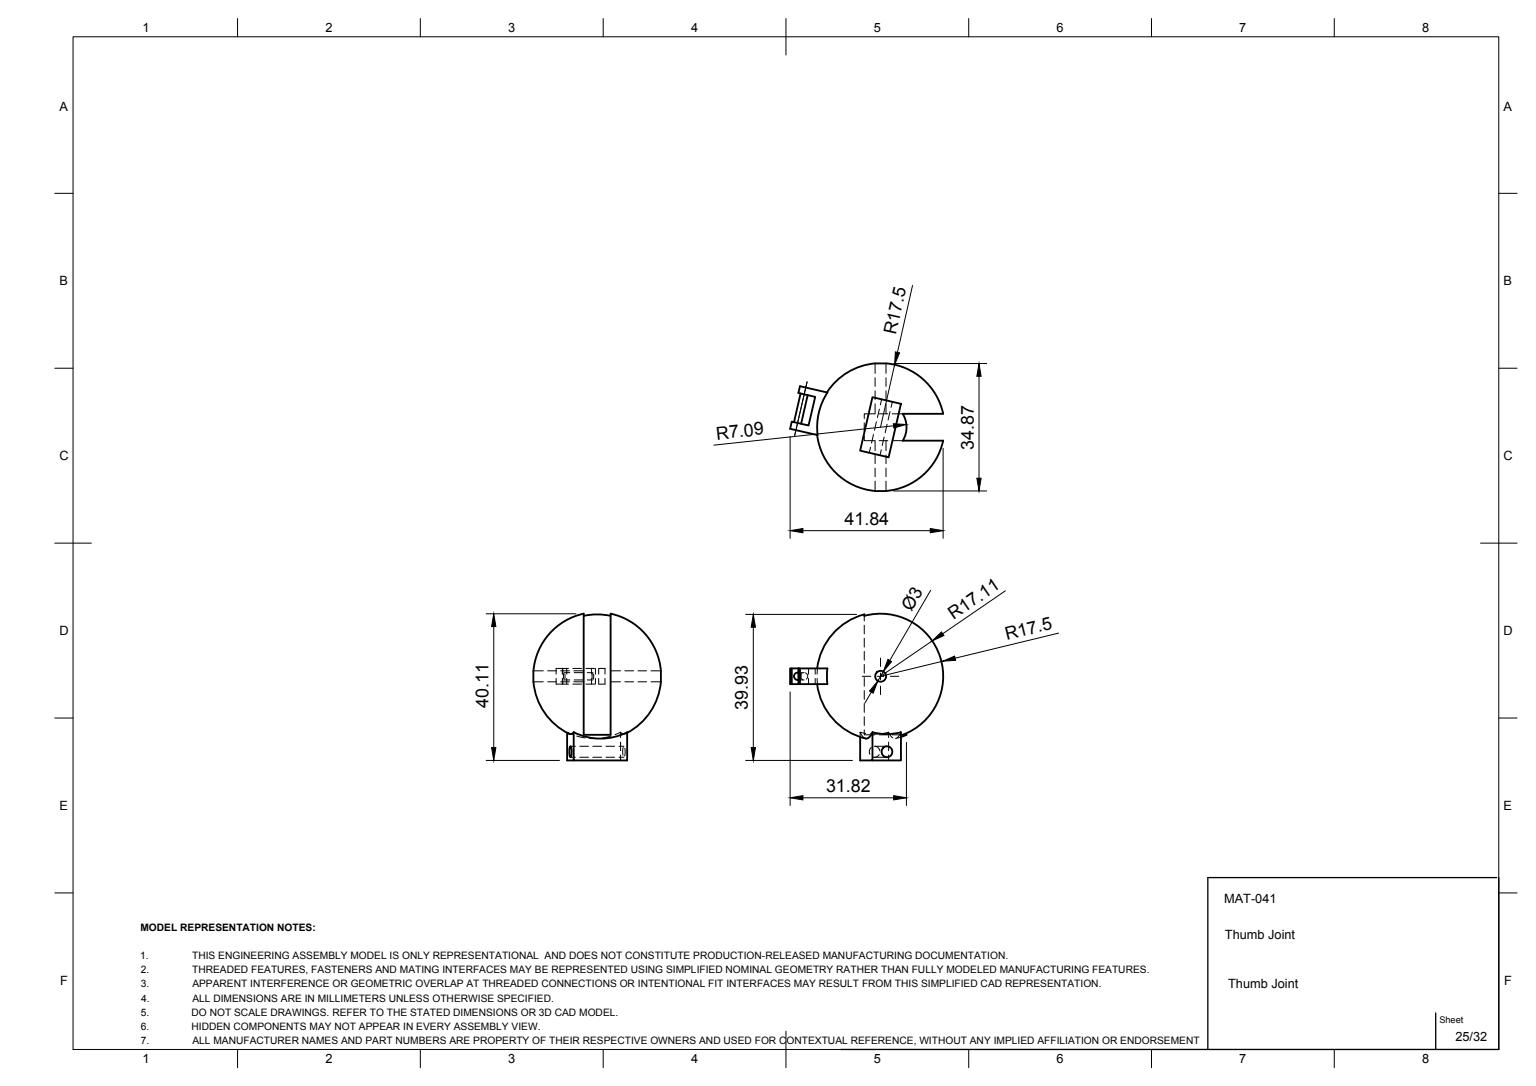
ISO-10303-21;
HEADER;
/* Generated by software containing ST-Developer
 * from STEP Tools, Inc. (www.steptools.com) 
 */

FILE_DESCRIPTION(
/* description */ ('STEP AP214'),
/* implementation_level */ '2;1');

FILE_NAME(
/* name */ 'Thumb Joint.step',
/* time_stamp */ '2026-11-14T21:57:47-08:00',
/* author */ (''),
/* organization */ (''),
/* preprocessor_version */ 'ST-DEVELOPER v20.2',
/* originating_system */ 'Autodesk Translation Framework v15.17.0.0',
/* authorisation */ '');

FILE_SCHEMA (('AUTOMOTIVE_DESIGN { 1 0 10303 214 3 1 1 }'));
ENDSEC;

DATA;
#10=MECHANICAL_DESIGN_GEOMETRIC_PRESENTATION_REPRESENTATION('',(#260),#13199);
#224=SHAPE_REPRESENTATION_RELATIONSHIP('SRR','None',#13296,#242);
#242=ADVANCED_BREP_SHAPE_REPRESENTATION('',(#278),#13192);
#260=STYLED_ITEM('',(#13410),#278);
#278=MANIFOLD_SOLID_BREP('Body1',#6855);
#354=FACE_BOUND('',#2551,.T.);
#355=FACE_BOUND('',#2552,.T.);
#356=FACE_BOUND('',#2556,.T.);
#357=FACE_BOUND('',#2559,.T.);
#358=FACE_BOUND('',#2562,.T.);
#359=FACE_BOUND('',#2565,.T.);
#360=FACE_BOUND('',#2574,.T.);
#361=FACE_BOUND('',#2576,.T.);
#543=PLANE('',#7648);
#544=PLANE('',#7649);
#545=PLANE('',#7650);
#546=PLANE('',#7651);
#547=PLANE('',#7652);
#548=PLANE('',#7653);
#549=PLANE('',#7654);
#550=PLANE('',#7655);
#551=PLANE('',#7656);
#552=PLANE('',#7657);
#553=PLANE('',#7658);
#554=PLANE('',#7659);
#555=PLANE('',#7660);
#556=PLANE('',#7661);
#557=PLANE('',#7662);
#558=PLANE('',#7663);
#559=PLANE('',#7664);
#560=PLANE('',#7665);
#980=LINE('',#12181,#1498);
#981=LINE('',#12187,#1499);
#982=LINE('',#12193,#1500);
#983=LINE('',#12199,#1501);
#984=LINE('',#12235,#1502);
#985=LINE('',#12237,#1503);
#986=LINE('',#12239,#1504);
#987=LINE('',#12240,#1505);
#988=LINE('',#12243,#1506);
#989=LINE('',#12245,#1507);
#990=LINE('',#12246,#1508);
#991=LINE('',#12249,#1509);
#992=LINE('',#12250,#1510);
#993=LINE('',#12253,#1511);
#994=LINE('',#12254,#1512);
#995=LINE('',#12256,#1513);
#996=LINE('',#12260,#1514);
#997=LINE('',#12261,#1515);
#998=LINE('',#12264,#1516);
#999=LINE('',#12265,#1517);
#1000=LINE('',#12267,#1518);
#1001=LINE('',#12272,#1519);
#1002=LINE('',#12273,#1520);
#1003=LINE('',#12274,#1521);
#1004=LINE('',#12276,#1522);
#1005=LINE('',#12278,#1523);
#1006=LINE('',#12279,#1524);
#1007=LINE('',#12282,#1525);
#1008=LINE('',#12283,#1526);
#1009=LINE('',#12286,#1527);
#1010=LINE('',#12288,#1528);
#1011=LINE('',#12290,#1529);
#1012=LINE('',#12291,#1530);
#1013=LINE('',#12292,#1531);
#1014=LINE('',#12295,#1532);
#1015=LINE('',#12297,#1533);
#1016=LINE('',#12298,#1534);
#1498=VECTOR('',#9321,1.);
#1499=VECTOR('',#9328,1.5);
#1500=VECTOR('',#9335,1.5);
#1501=VECTOR('',#9342,1.5);
#1502=VECTOR('',#9381,1000.);
#1503=VECTOR('',#9382,1000.);
#1504=VECTOR('',#9383,1000.);
#1505=VECTOR('',#9384,1000.);
#1506=VECTOR('',#9387,1000.);
#1507=VECTOR('',#9388,1000.);
#1508=VECTOR('',#9389,1000.);
#1509=VECTOR('',#9392,1000.);
#1510=VECTOR('',#9393,1000.);
#1511=VECTOR('',#9396,1000.);
#1512=VECTOR('',#9397,1000.);
#1513=VECTOR('',#9400,1000.);
#1514=VECTOR('',#9405,1000.);
#1515=VECTOR('',#9406,1000.);
#1516=VECTOR('',#9409,1000.);
#1517=VECTOR('',#9410,1000.);
#1518=VECTOR('',#9413,1000.);
#1519=VECTOR('',#9418,1000.);
#1520=VECTOR('',#9419,1000.);
#1521=VECTOR('',#9420,1000.);
#1522=VECTOR('',#9421,1000.);
#1523=VECTOR('',#9422,1000.);
#1524=VECTOR('',#9423,1000.);
#1525=VECTOR('',#9426,1000.);
#1526=VECTOR('',#9427,1000.);
#1527=VECTOR('',#9430,1000.);
#1528=VECTOR('',#9431,1000.);
#1529=VECTOR('',#9432,1000.);
#1530=VECTOR('',#9433,1000.);
#1531=VECTOR('',#9434,1000.);
#1532=VECTOR('',#9439,1000.);
#1533=VECTOR('',#9442,1000.);
#1534=VECTOR('',#9443,1000.);
#1757=CYLINDRICAL_SURFACE('',#7619,1.);
#1758=CYLINDRICAL_SURFACE('',#7622,1.5);
#1759=CYLINDRICAL_SURFACE('',#7625,1.5);
#1760=CYLINDRICAL_SURFACE('',#7628,1.5);
#1799=SPHERICAL_SURFACE('',#7631,17.5);
#2085=FACE_OUTER_BOUND('',#2546,.T.);
#2086=FACE_OUTER_BOUND('',#2547,.T.);
#2087=FACE_OUTER_BOUND('',#2548,.T.);
#2088=FACE_OUTER_BOUND('',#2549,.T.);
#2089=FACE_OUTER_BOUND('',#2550,.T.);
#2090=FACE_OUTER_BOUND('',#2553,.T.);
#2091=FACE_OUTER_BOUND('',#2554,.T.);
#2092=FACE_OUTER_BOUND('',#2555,.T.);
#2093=FACE_OUTER_BOUND('',#2557,.T.);
#2094=FACE_OUTER_BOUND('',#2558,.T.);
#2095=FACE_OUTER_BOUND('',#2560,.T.);
#2096=FACE_OUTER_BOUND('',#2561,.T.);
#2097=FACE_OUTER_BOUND('',#2563,.T.);
#2098=FACE_OUTER_BOUND('',#2564,.T.);
#2099=FACE_OUTER_BOUND('',#2566,.T.);
#2100=FACE_OUTER_BOUND('',#2567,.T.);
#2101=FACE_OUTER_BOUND('',#2568,.T.);
#2102=FACE_OUTER_BOUND('',#2569,.T.);
#2103=FACE_OUTER_BOUND('',#2570,.T.);
#2104=FACE_OUTER_BOUND('',#2571,.T.);
#2105=FACE_OUTER_BOUND('',#2572,.T.);
#2106=FACE_OUTER_BOUND('',#2573,.T.);
#2107=FACE_OUTER_BOUND('',#2575,.T.);
#2546=EDGE_LOOP('',(#5910,#5911,#5912,#5913));
#2547=EDGE_LOOP('',(#5914,#5915,#5916,#5917));
#2548=EDGE_LOOP('',(#5918,#5919,#5920,#5921));
#2549=EDGE_LOOP('',(#5922,#5923,#5924,#5925));
#2550=EDGE_LOOP('',(#5926,#5927,#5928,#5929,#5930,#5931,#5932,#5933,#5934,
#5935,#5936,#5937));
#2551=EDGE_LOOP('',(#5938,#5939,#5940,#5941));
#2552=EDGE_LOOP('',(#5942,#5943,#5944,#5945));
#2553=EDGE_LOOP('',(#5946,#5947,#5948,#5949));
#2554=EDGE_LOOP('',(#5950,#5951,#5952,#5953));
#2555=EDGE_LOOP('',(#5954,#5955,#5956,#5957));
#2556=EDGE_LOOP('',(#5958));
#2557=EDGE_LOOP('',(#5959,#5960,#5961,#5962));
#2558=EDGE_LOOP('',(#5963,#5964,#5965,#5966));
#2559=EDGE_LOOP('',(#5967));
#2560=EDGE_LOOP('',(#5968,#5969,#5970,#5971));
#2561=EDGE_LOOP('',(#5972,#5973,#5974,#5975));
#2562=EDGE_LOOP('',(#5976));
#2563=EDGE_LOOP('',(#5977,#5978,#5979,#5980));
#2564=EDGE_LOOP('',(#5981,#5982,#5983,#5984));
#2565=EDGE_LOOP('',(#5985));
#2566=EDGE_LOOP('',(#5986,#5987,#5988,#5989));
#2567=EDGE_LOOP('',(#5990,#5991,#5992,#5993,#5994,#5995,#5996,#5997));
#2568=EDGE_LOOP('',(#5998,#5999,#6000,#6001));
#2569=EDGE_LOOP('',(#6002,#6003,#6004,#6005,#6006,#6007,#6008,#6009));
#2570=EDGE_LOOP('',(#6010,#6011,#6012,#6013));
#2571=EDGE_LOOP('',(#6014,#6015,#6016,#6017));
#2572=EDGE_LOOP('',(#6018,#6019,#6020,#6021));
#2573=EDGE_LOOP('',(#6022,#6023,#6024,#6025));
#2574=EDGE_LOOP('',(#6026));
#2575=EDGE_LOOP('',(#6027,#6028,#6029,#6030));
#2576=EDGE_LOOP('',(#6031));
#2915=CIRCLE('',#7620,1.);
#2916=CIRCLE('',#7621,1.);
#2917=CIRCLE('',#7623,1.5);
#2918=CIRCLE('',#7624,1.5);
#2919=CIRCLE('',#7626,1.5);
#2920=CIRCLE('',#7627,1.5);
#2921=CIRCLE('',#7629,1.5);
#2922=CIRCLE('',#7630,1.5);
#2923=CIRCLE('',#7632,17.5);
#2924=CIRCLE('',#7633,17.1097742533325);
#2925=CIRCLE('',#7634,7.08872343937892);
#2926=CIRCLE('',#7635,17.1097742533325);
#2927=CIRCLE('',#7636,17.5);
#2928=CIRCLE('',#7637,17.1097742533325);
#2929=CIRCLE('',#7638,16.9253361239603);
#2930=CIRCLE('',#7639,17.1097742533325);
#2931=CIRCLE('',#7640,17.3675981074726);
#2932=CIRCLE('',#7641,16.4471056942753);
#2933=CIRCLE('',#7642,17.3675981074726);
#2934=CIRCLE('',#7643,16.4471056942753);
#2935=CIRCLE('',#7644,17.0367250374008);
#2936=CIRCLE('',#7645,15.8113883008419);
#2937=CIRCLE('',#7646,17.0367250374008);
#2938=CIRCLE('',#7647,15.8113883008419);
#3439=VERTEX_POINT('',#12178);
#3440=VERTEX_POINT('',#12180);
#3441=VERTEX_POINT('',#12184);
#3442=VERTEX_POINT('',#12186);
#3443=VERTEX_POINT('',#12190);
#3444=VERTEX_POINT('',#12192);
#3445=VERTEX_POINT('',#12196);
#3446=VERTEX_POINT('',#12198);
#3447=VERTEX_POINT('',#12202);
#3448=VERTEX_POINT('',#12204);
#3449=VERTEX_POINT('',#12206);
#3450=VERTEX_POINT('',#12208);
#3451=VERTEX_POINT('',#12211);
#3452=VERTEX_POINT('',#12213);
#3453=VERTEX_POINT('',#12216);
#3454=VERTEX_POINT('',#12217);
#3455=VERTEX_POINT('',#12219);
#3456=VERTEX_POINT('',#12221);
#3457=VERTEX_POINT('',#12224);
#3458=VERTEX_POINT('',#12225);
#3459=VERTEX_POINT('',#12227);
#3460=VERTEX_POINT('',#12229);
#3461=VERTEX_POINT('',#12233);
#3462=VERTEX_POINT('',#12234);
#3463=VERTEX_POINT('',#12236);
#3464=VERTEX_POINT('',#12238);
#3465=VERTEX_POINT('',#12242);
#3466=VERTEX_POINT('',#12244);
#3467=VERTEX_POINT('',#12248);
#3468=VERTEX_POINT('',#12252);
#3469=VERTEX_POINT('',#12259);
#3470=VERTEX_POINT('',#12263);
#3471=VERTEX_POINT('',#12270);
#3472=VERTEX_POINT('',#12271);
#3473=VERTEX_POINT('',#12275);
#3474=VERTEX_POINT('',#12277);
#3475=VERTEX_POINT('',#12281);
#3476=VERTEX_POINT('',#12285);
#3477=VERTEX_POINT('',#12287);
#3478=VERTEX_POINT('',#12289);
#4292=EDGE_CURVE('',#3439,#3439,#2915,.T.);
#4293=EDGE_CURVE('',#3439,#3440,#980,.T.);
#4294=EDGE_CURVE('',#3440,#3440,#2916,.T.);
#4295=EDGE_CURVE('',#3441,#3441,#2917,.T.);
#4296=EDGE_CURVE('',#3441,#3442,#981,.T.);
#4297=EDGE_CURVE('',#3442,#3442,#2918,.T.);
#4298=EDGE_CURVE('',#3443,#3443,#2919,.T.);
#4299=EDGE_CURVE('',#3443,#3444,#982,.T.);
#4300=EDGE_CURVE('',#3444,#3444,#2920,.T.);
#4301=EDGE_CURVE('',#3445,#3445,#2921,.T.);
#4302=EDGE_CURVE('',#3445,#3446,#983,.T.);
#4303=EDGE_CURVE('',#3446,#3446,#2922,.T.);
#4304=EDGE_CURVE('',#3444,#3447,#2923,.T.);
#4305=EDGE_CURVE('',#3448,#3447,#2924,.T.);
#4306=EDGE_CURVE('',#3449,#3448,#2925,.T.);
#4307=EDGE_CURVE('',#3450,#3449,#2926,.T.);
#4308=EDGE_CURVE('',#3450,#3445,#2927,.T.);
#4309=EDGE_CURVE('',#3451,#3450,#2928,.T.);
#4310=EDGE_CURVE('',#3452,#3451,#2929,.T.);
#4311=EDGE_CURVE('',#3447,#3452,#2930,.T.);
#4312=EDGE_CURVE('',#3453,#3454,#2931,.T.);
#4313=EDGE_CURVE('',#3455,#3453,#2932,.T.);
#4314=EDGE_CURVE('',#3456,#3455,#2933,.T.);
#4315=EDGE_CURVE('',#3454,#3456,#2934,.T.);
#4316=EDGE_CURVE('',#3457,#3458,#2935,.T.);
#4317=EDGE_CURVE('',#3458,#3459,#2936,.T.);
#4318=EDGE_CURVE('',#3460,#3459,#2937,.T.);
#4319=EDGE_CURVE('',#3457,#3460,#2938,.T.);
#4320=EDGE_CURVE('',#3461,#3462,#984,.T.);
#4321=EDGE_CURVE('',#3461,#3463,#985,.T.);
#4322=EDGE_CURVE('',#3463,#3464,#986,.T.);
#4323=EDGE_CURVE('',#3464,#3462,#987,.T.);
#4324=EDGE_CURVE('',#3465,#3457,#988,.T.);
#4325=EDGE_CURVE('',#3465,#3466,#989,.T.);
#4326=EDGE_CURVE('',#3466,#3458,#990,.T.);
#4327=EDGE_CURVE('',#3467,#3460,#991,.T.);
#4328=EDGE_CURVE('',#3465,#3467,#992,.T.);
#4329=EDGE_CURVE('',#3468,#3459,#993,.T.);
#4330=EDGE_CURVE('',#3467,#3468,#994,.T.);
#4331=EDGE_CURVE('',#3466,#3468,#995,.T.);
#4332=EDGE_CURVE('',#3452,#3469,#996,.T.);
#4333=EDGE_CURVE('',#3448,#3469,#997,.T.);
#4334=EDGE_CURVE('',#3451,#3470,#998,.T.);
#4335=EDGE_CURVE('',#3469,#3470,#999,.T.);
#4336=EDGE_CURVE('',#3470,#3449,#1000,.T.);
#4337=EDGE_CURVE('',#3471,#3472,#1001,.T.);
#4338=EDGE_CURVE('',#3472,#3462,#1002,.T.);
#4339=EDGE_CURVE('',#3464,#3456,#1003,.T.);
#4340=EDGE_CURVE('',#3473,#3455,#1004,.T.);
#4341=EDGE_CURVE('',#3474,#3473,#1005,.T.);
#4342=EDGE_CURVE('',#3474,#3471,#1006,.T.);
#4343=EDGE_CURVE('',#3475,#3453,#1007,.T.);
#4344=EDGE_CURVE('',#3473,#3475,#1008,.T.);
#4345=EDGE_CURVE('',#3476,#3461,#1009,.T.);
#4346=EDGE_CURVE('',#3477,#3476,#1010,.T.);
#4347=EDGE_CURVE('',#3478,#3477,#1011,.T.);
#4348=EDGE_CURVE('',#3475,#3478,#1012,.T.);
#4349=EDGE_CURVE('',#3463,#3454,#1013,.T.);
#4350=EDGE_CURVE('',#3474,#3478,#1014,.T.);
#4351=EDGE_CURVE('',#3471,#3477,#1015,.T.);
#4352=EDGE_CURVE('',#3472,#3476,#1016,.T.);
#5910=ORIENTED_EDGE('',*,*,#4292,.F.);
#5911=ORIENTED_EDGE('',*,*,#4293,.T.);
#5912=ORIENTED_EDGE('',*,*,#4294,.T.);
#5913=ORIENTED_EDGE('',*,*,#4293,.F.);
#5914=ORIENTED_EDGE('',*,*,#4295,.F.);
#5915=ORIENTED_EDGE('',*,*,#4296,.T.);
#5916=ORIENTED_EDGE('',*,*,#4297,.T.);
#5917=ORIENTED_EDGE('',*,*,#4296,.F.);
#5918=ORIENTED_EDGE('',*,*,#4298,.F.);
#5919=ORIENTED_EDGE('',*,*,#4299,.T.);
#5920=ORIENTED_EDGE('',*,*,#4300,.T.);
#5921=ORIENTED_EDGE('',*,*,#4299,.F.);
#5922=ORIENTED_EDGE('',*,*,#4301,.T.);
#5923=ORIENTED_EDGE('',*,*,#4302,.T.);
#5924=ORIENTED_EDGE('',*,*,#4303,.F.);
#5925=ORIENTED_EDGE('',*,*,#4302,.F.);
#5926=ORIENTED_EDGE('',*,*,#4300,.F.);
#5927=ORIENTED_EDGE('',*,*,#4304,.T.);
#5928=ORIENTED_EDGE('',*,*,#4305,.F.);
#5929=ORIENTED_EDGE('',*,*,#4306,.F.);
#5930=ORIENTED_EDGE('',*,*,#4307,.F.);
#5931=ORIENTED_EDGE('',*,*,#4308,.T.);
#5932=ORIENTED_EDGE('',*,*,#4301,.F.);
#5933=ORIENTED_EDGE('',*,*,#4308,.F.);
#5934=ORIENTED_EDGE('',*,*,#4309,.F.);
#5935=ORIENTED_EDGE('',*,*,#4310,.F.);
#5936=ORIENTED_EDGE('',*,*,#4311,.F.);
#5937=ORIENTED_EDGE('',*,*,#4304,.F.);
#5938=ORIENTED_EDGE('',*,*,#4312,.F.);
#5939=ORIENTED_EDGE('',*,*,#4313,.F.);
#5940=ORIENTED_EDGE('',*,*,#4314,.F.);
#5941=ORIENTED_EDGE('',*,*,#4315,.F.);
#5942=ORIENTED_EDGE('',*,*,#4316,.T.);
#5943=ORIENTED_EDGE('',*,*,#4317,.T.);
#5944=ORIENTED_EDGE('',*,*,#4318,.F.);
#5945=ORIENTED_EDGE('',*,*,#4319,.F.);
#5946=ORIENTED_EDGE('',*,*,#4320,.F.);
#5947=ORIENTED_EDGE('',*,*,#4321,.T.);
#5948=ORIENTED_EDGE('',*,*,#4322,.T.);
#5949=ORIENTED_EDGE('',*,*,#4323,.T.);
#5950=ORIENTED_EDGE('',*,*,#4316,.F.);
#5951=ORIENTED_EDGE('',*,*,#4324,.F.);
#5952=ORIENTED_EDGE('',*,*,#4325,.T.);
#5953=ORIENTED_EDGE('',*,*,#4326,.T.);
#5954=ORIENTED_EDGE('',*,*,#4324,.T.);
#5955=ORIENTED_EDGE('',*,*,#4319,.T.);
#5956=ORIENTED_EDGE('',*,*,#4327,.F.);
#5957=ORIENTED_EDGE('',*,*,#4328,.F.);
#5958=ORIENTED_EDGE('',*,*,#4295,.T.);
#5959=ORIENTED_EDGE('',*,*,#4327,.T.);
#5960=ORIENTED_EDGE('',*,*,#4318,.T.);
#5961=ORIENTED_EDGE('',*,*,#4329,.F.);
#5962=ORIENTED_EDGE('',*,*,#4330,.F.);
#5963=ORIENTED_EDGE('',*,*,#4317,.F.);
#5964=ORIENTED_EDGE('',*,*,#4326,.F.);
#5965=ORIENTED_EDGE('',*,*,#4331,.T.);
#5966=ORIENTED_EDGE('',*,*,#4329,.T.);
#5967=ORIENTED_EDGE('',*,*,#4297,.F.);
#5968=ORIENTED_EDGE('',*,*,#4325,.F.);
#5969=ORIENTED_EDGE('',*,*,#4328,.T.);
#5970=ORIENTED_EDGE('',*,*,#4330,.T.);
#5971=ORIENTED_EDGE('',*,*,#4331,.F.);
#5972=ORIENTED_EDGE('',*,*,#4305,.T.);
#5973=ORIENTED_EDGE('',*,*,#4311,.T.);
#5974=ORIENTED_EDGE('',*,*,#4332,.T.);
#5975=ORIENTED_EDGE('',*,*,#4333,.F.);
#5976=ORIENTED_EDGE('',*,*,#4298,.T.);
#5977=ORIENTED_EDGE('',*,*,#4310,.T.);
#5978=ORIENTED_EDGE('',*,*,#4334,.T.);
#5979=ORIENTED_EDGE('',*,*,#4335,.F.);
#5980=ORIENTED_EDGE('',*,*,#4332,.F.);
#5981=ORIENTED_EDGE('',*,*,#4309,.T.);
#5982=ORIENTED_EDGE('',*,*,#4307,.T.);
#5983=ORIENTED_EDGE('',*,*,#4336,.F.);
#5984=ORIENTED_EDGE('',*,*,#4334,.F.);
#5985=ORIENTED_EDGE('',*,*,#4303,.T.);
#5986=ORIENTED_EDGE('',*,*,#4306,.T.);
#5987=ORIENTED_EDGE('',*,*,#4333,.T.);
#5988=ORIENTED_EDGE('',*,*,#4335,.T.);
#5989=ORIENTED_EDGE('',*,*,#4336,.T.);
#5990=ORIENTED_EDGE('',*,*,#4337,.T.);
#5991=ORIENTED_EDGE('',*,*,#4338,.T.);
#5992=ORIENTED_EDGE('',*,*,#4323,.F.);
#5993=ORIENTED_EDGE('',*,*,#4339,.T.);
#5994=ORIENTED_EDGE('',*,*,#4314,.T.);
#5995=ORIENTED_EDGE('',*,*,#4340,.F.);
#5996=ORIENTED_EDGE('',*,*,#4341,.F.);
#5997=ORIENTED_EDGE('',*,*,#4342,.T.);
#5998=ORIENTED_EDGE('',*,*,#4340,.T.);
#5999=ORIENTED_EDGE('',*,*,#4313,.T.);
#6000=ORIENTED_EDGE('',*,*,#4343,.F.);
#6001=ORIENTED_EDGE('',*,*,#4344,.F.);
#6002=ORIENTED_EDGE('',*,*,#4321,.F.);
#6003=ORIENTED_EDGE('',*,*,#4345,.F.);
#6004=ORIENTED_EDGE('',*,*,#4346,.F.);
#6005=ORIENTED_EDGE('',*,*,#4347,.F.);
#6006=ORIENTED_EDGE('',*,*,#4348,.F.);
#6007=ORIENTED_EDGE('',*,*,#4343,.T.);
#6008=ORIENTED_EDGE('',*,*,#4312,.T.);
#6009=ORIENTED_EDGE('',*,*,#4349,.F.);
#6010=ORIENTED_EDGE('',*,*,#4349,.T.);
#6011=ORIENTED_EDGE('',*,*,#4315,.T.);
#6012=ORIENTED_EDGE('',*,*,#4339,.F.);
#6013=ORIENTED_EDGE('',*,*,#4322,.F.);
#6014=ORIENTED_EDGE('',*,*,#4350,.F.);
#6015=ORIENTED_EDGE('',*,*,#4341,.T.);
#6016=ORIENTED_EDGE('',*,*,#4344,.T.);
#6017=ORIENTED_EDGE('',*,*,#4348,.T.);
#6018=ORIENTED_EDGE('',*,*,#4351,.T.);
#6019=ORIENTED_EDGE('',*,*,#4346,.T.);
#6020=ORIENTED_EDGE('',*,*,#4352,.F.);
#6021=ORIENTED_EDGE('',*,*,#4337,.F.);
#6022=ORIENTED_EDGE('',*,*,#4352,.T.);
#6023=ORIENTED_EDGE('',*,*,#4345,.T.);
#6024=ORIENTED_EDGE('',*,*,#4320,.T.);
#6025=ORIENTED_EDGE('',*,*,#4338,.F.);
#6026=ORIENTED_EDGE('',*,*,#4292,.T.);
#6027=ORIENTED_EDGE('',*,*,#4350,.T.);
#6028=ORIENTED_EDGE('',*,*,#4347,.T.);
#6029=ORIENTED_EDGE('',*,*,#4351,.F.);
#6030=ORIENTED_EDGE('',*,*,#4342,.F.);
#6031=ORIENTED_EDGE('',*,*,#4294,.F.);
#6737=ADVANCED_FACE('',(#2085),#1757,.T.);
#6738=ADVANCED_FACE('',(#2086),#1758,.F.);
#6739=ADVANCED_FACE('',(#2087),#1759,.F.);
#6740=ADVANCED_FACE('',(#2088),#1760,.F.);
#6741=ADVANCED_FACE('',(#2089,#354,#355),#1799,.T.);
#6742=ADVANCED_FACE('',(#2090),#543,.T.);
#6743=ADVANCED_FACE('',(#2091),#544,.T.);
#6744=ADVANCED_FACE('',(#2092,#356),#545,.F.);
#6745=ADVANCED_FACE('',(#2093),#546,.F.);
#6746=ADVANCED_FACE('',(#2094,#357),#547,.T.);
#6747=ADVANCED_FACE('',(#2095),#548,.F.);
#6748=ADVANCED_FACE('',(#2096,#358),#549,.T.);
#6749=ADVANCED_FACE('',(#2097),#550,.T.);
#6750=ADVANCED_FACE('',(#2098,#359),#551,.T.);
#6751=ADVANCED_FACE('',(#2099),#552,.T.);
#6752=ADVANCED_FACE('',(#2100),#553,.F.);
#6753=ADVANCED_FACE('',(#2101),#554,.F.);
#6754=ADVANCED_FACE('',(#2102),#555,.F.);
#6755=ADVANCED_FACE('',(#2103),#556,.F.);
#6756=ADVANCED_FACE('',(#2104),#557,.T.);
#6757=ADVANCED_FACE('',(#2105),#558,.F.);
#6758=ADVANCED_FACE('',(#2106,#360),#559,.F.);
#6759=ADVANCED_FACE('',(#2107,#361),#560,.F.);
#6855=CLOSED_SHELL('',(#6737,#6738,#6739,#6740,#6741,#6742,#6743,#6744,
#6745,#6746,#6747,#6748,#6749,#6750,#6751,#6752,#6753,#6754,#6755,#6756,
#6757,#6758,#6759));
#7618=AXIS2_PLACEMENT_3D('',#12176,#9315,#9316);
#7619=AXIS2_PLACEMENT_3D('',#12177,#9317,#9318);
#7620=AXIS2_PLACEMENT_3D('',#12179,#9319,#9320);
#7621=AXIS2_PLACEMENT_3D('',#12182,#9322,#9323);
#7622=AXIS2_PLACEMENT_3D('',#12183,#9324,#9325);
#7623=AXIS2_PLACEMENT_3D('',#12185,#9326,#9327);
#7624=AXIS2_PLACEMENT_3D('',#12188,#9329,#9330);
#7625=AXIS2_PLACEMENT_3D('',#12189,#9331,#9332);
#7626=AXIS2_PLACEMENT_3D('',#12191,#9333,#9334);
#7627=AXIS2_PLACEMENT_3D('',#12194,#9336,#9337);
#7628=AXIS2_PLACEMENT_3D('',#12195,#9338,#9339);
#7629=AXIS2_PLACEMENT_3D('',#12197,#9340,#9341);
#7630=AXIS2_PLACEMENT_3D('',#12200,#9343,#9344);
#7631=AXIS2_PLACEMENT_3D('',#12201,#9345,#9346);
#7632=AXIS2_PLACEMENT_3D('',#12203,#9347,#9348);
#7633=AXIS2_PLACEMENT_3D('',#12205,#9349,#9350);
#7634=AXIS2_PLACEMENT_3D('',#12207,#9351,#9352);
#7635=AXIS2_PLACEMENT_3D('',#12209,#9353,#9354);
#7636=AXIS2_PLACEMENT_3D('',#12210,#9355,#9356);
#7637=AXIS2_PLACEMENT_3D('',#12212,#9357,#9358);
#7638=AXIS2_PLACEMENT_3D('',#12214,#9359,#9360);
#7639=AXIS2_PLACEMENT_3D('',#12215,#9361,#9362);
#7640=AXIS2_PLACEMENT_3D('',#12218,#9363,#9364);
#7641=AXIS2_PLACEMENT_3D('',#12220,#9365,#9366);
#7642=AXIS2_PLACEMENT_3D('',#12222,#9367,#9368);
#7643=AXIS2_PLACEMENT_3D('',#12223,#9369,#9370);
#7644=AXIS2_PLACEMENT_3D('',#12226,#9371,#9372);
#7645=AXIS2_PLACEMENT_3D('',#12228,#9373,#9374);
#7646=AXIS2_PLACEMENT_3D('',#12230,#9375,#9376);
#7647=AXIS2_PLACEMENT_3D('',#12231,#9377,#9378);
#7648=AXIS2_PLACEMENT_3D('',#12232,#9379,#9380);
#7649=AXIS2_PLACEMENT_3D('',#12241,#9385,#9386);
#7650=AXIS2_PLACEMENT_3D('',#12247,#9390,#9391);
#7651=AXIS2_PLACEMENT_3D('',#12251,#9394,#9395);
#7652=AXIS2_PLACEMENT_3D('',#12255,#9398,#9399);
#7653=AXIS2_PLACEMENT_3D('',#12257,#9401,#9402);
#7654=AXIS2_PLACEMENT_3D('',#12258,#9403,#9404);
#7655=AXIS2_PLACEMENT_3D('',#12262,#9407,#9408);
#7656=AXIS2_PLACEMENT_3D('',#12266,#9411,#9412);
#7657=AXIS2_PLACEMENT_3D('',#12268,#9414,#9415);
#7658=AXIS2_PLACEMENT_3D('',#12269,#9416,#9417);
#7659=AXIS2_PLACEMENT_3D('',#12280,#9424,#9425);
#7660=AXIS2_PLACEMENT_3D('',#12284,#9428,#9429);
#7661=AXIS2_PLACEMENT_3D('',#12293,#9435,#9436);
#7662=AXIS2_PLACEMENT_3D('',#12294,#9437,#9438);
#7663=AXIS2_PLACEMENT_3D('',#12296,#9440,#9441);
#7664=AXIS2_PLACEMENT_3D('',#12299,#9444,#9445);
#7665=AXIS2_PLACEMENT_3D('',#12300,#9446,#9447);
#9315=DIRECTION('axis',(0.,0.,1.));
#9316=DIRECTION('refdir',(1.,0.,0.));
#9317=DIRECTION('center_axis',(0.,-0.224951054343868,0.974370064785235));
#9318=DIRECTION('ref_axis',(0.,-0.974370064785235,-0.224951054343868));
#9319=DIRECTION('center_axis',(0.,-0.224951054343868,0.974370064785235));
#9320=DIRECTION('ref_axis',(0.,-0.974370064785235,-0.224951054343868));
#9321=DIRECTION('',(0.,0.224951054343868,-0.974370064785235));
#9322=DIRECTION('center_axis',(0.,-0.224951054343868,0.974370064785235));
#9323=DIRECTION('ref_axis',(0.,0.974370064785235,0.224951054343868));
#9324=DIRECTION('center_axis',(0.,-0.224951054343865,0.974370064785235));
#9325=DIRECTION('ref_axis',(0.,-0.974370064785235,-0.224951054343865));
#9326=DIRECTION('center_axis',(0.,-0.224951054343865,0.974370064785235));
#9327=DIRECTION('ref_axis',(0.,-0.974370064785235,-0.224951054343865));
#9328=DIRECTION('',(0.,-0.224951054343865,0.974370064785235));
#9329=DIRECTION('center_axis',(0.,-0.224951054343865,0.974370064785235));
#9330=DIRECTION('ref_axis',(0.,-0.974370064785235,-0.224951054343865));
#9331=DIRECTION('center_axis',(0.,0.,-1.));
#9332=DIRECTION('ref_axis',(-1.,0.,0.));
#9333=DIRECTION('center_axis',(0.,1.1019100660974E-16,-1.));
#9334=DIRECTION('ref_axis',(0.,-1.,-1.1019100660974E-16));
#9335=DIRECTION('',(0.,0.,-1.));
#9336=DIRECTION('center_axis',(0.,0.,-1.));
#9337=DIRECTION('ref_axis',(1.,0.,0.));
#9338=DIRECTION('center_axis',(0.,0.,-1.));
#9339=DIRECTION('ref_axis',(-1.,0.,0.));
#9340=DIRECTION('center_axis',(0.,0.,1.));
#9341=DIRECTION('ref_axis',(-1.,0.,0.));
#9342=DIRECTION('',(0.,0.,-1.));
#9343=DIRECTION('center_axis',(0.,-9.18258388414501E-17,1.));
#9344=DIRECTION('ref_axis',(0.,1.,9.18258388414501E-17));
#9345=DIRECTION('center_axis',(-6.12323399573677E-17,0.,-1.));
#9346=DIRECTION('ref_axis',(-1.,0.,0.));
#9347=DIRECTION('center_axis',(-1.26882631385732E-16,-1.,0.));
#9348=DIRECTION('ref_axis',(1.,-1.26882631385732E-16,0.));
#9349=DIRECTION('center_axis',(0.,-1.1019100660974E-16,1.));
#9350=DIRECTION('ref_axis',(0.,-1.,-1.1019100660974E-16));
#9351=DIRECTION('center_axis',(1.,0.,0.));
#9352=DIRECTION('ref_axis',(0.,0.,-1.));
#9353=DIRECTION('center_axis',(0.,9.18258388414501E-17,-1.));
#9354=DIRECTION('ref_axis',(0.,1.,9.18258388414501E-17));
#9355=DIRECTION('center_axis',(-1.26882631385732E-16,-1.,0.));
#9356=DIRECTION('ref_axis',(1.,-1.26882631385732E-16,0.));
#9357=DIRECTION('center_axis',(0.,9.18258388414501E-17,-1.));
#9358=DIRECTION('ref_axis',(0.,1.,9.18258388414501E-17));
#9359=DIRECTION('center_axis',(0.,-1.,0.));
#9360=DIRECTION('ref_axis',(0.,0.,-1.));
#9361=DIRECTION('center_axis',(0.,-1.1019100660974E-16,1.));
#9362=DIRECTION('ref_axis',(0.,-1.,-1.1019100660974E-16));
#9363=DIRECTION('center_axis',(1.,0.,0.));
#9364=DIRECTION('ref_axis',(0.,0.,-1.));
#9365=DIRECTION('center_axis',(0.,-0.224951054343868,0.974370064785235));
#9366=DIRECTION('ref_axis',(0.,-0.974370064785235,-0.224951054343868));
#9367=DIRECTION('center_axis',(-1.,0.,0.));
#9368=DIRECTION('ref_axis',(0.,0.,1.));
#9369=DIRECTION('center_axis',(0.,0.224951054343868,-0.974370064785235));
#9370=DIRECTION('ref_axis',(0.,0.974370064785235,0.224951054343868));
#9371=DIRECTION('center_axis',(0.,0.974370064785235,0.224951054343868));
#9372=DIRECTION('ref_axis',(0.,-0.224951054343868,0.974370064785235));
#9373=DIRECTION('center_axis',(0.,-0.224951054343865,0.974370064785235));
#9374=DIRECTION('ref_axis',(0.,-0.974370064785235,-0.224951054343865));
#9375=DIRECTION('center_axis',(0.,0.974370064785235,0.224951054343868));
#9376=DIRECTION('ref_axis',(0.,-0.224951054343868,0.974370064785235));
#9377=DIRECTION('center_axis',(0.,-0.224951054343865,0.974370064785235));
#9378=DIRECTION('ref_axis',(0.,-0.974370064785235,-0.224951054343865));
#9379=DIRECTION('center_axis',(0.,0.974370064785235,0.224951054343868));
#9380=DIRECTION('ref_axis',(0.,-0.224951054343868,0.974370064785235));
#9381=DIRECTION('',(1.,0.,0.));
#9382=DIRECTION('',(0.,-0.224951054343868,0.974370064785235));
#9383=DIRECTION('',(1.,0.,0.));
#9384=DIRECTION('',(0.,0.224951054343868,-0.974370064785235));
#9385=DIRECTION('center_axis',(0.,0.974370064785235,0.224951054343868));
#9386=DIRECTION('ref_axis',(0.,-0.224951054343868,0.974370064785235));
#9387=DIRECTION('',(1.,0.,0.));
#9388=DIRECTION('',(0.,-0.224951054343868,0.974370064785235));
#9389=DIRECTION('',(1.,0.,0.));
#9390=DIRECTION('center_axis',(0.,-0.224951054343865,0.974370064785235));
#9391=DIRECTION('ref_axis',(0.,-0.974370064785235,-0.224951054343865));
#9392=DIRECTION('',(1.,0.,0.));
#9393=DIRECTION('',(0.,-0.974370064785235,-0.224951054343865));
#9394=DIRECTION('center_axis',(0.,0.974370064785235,0.224951054343868));
#9395=DIRECTION('ref_axis',(0.,-0.224951054343868,0.974370064785235));
#9396=DIRECTION('',(1.,0.,0.));
#9397=DIRECTION('',(0.,-0.224951054343868,0.974370064785235));
#9398=DIRECTION('center_axis',(0.,-0.224951054343865,0.974370064785235));
#9399=DIRECTION('ref_axis',(0.,-0.974370064785235,-0.224951054343865));
#9400=DIRECTION('',(0.,-0.974370064785235,-0.224951054343865));
#9401=DIRECTION('center_axis',(1.,0.,0.));
#9402=DIRECTION('ref_axis',(0.,0.,-1.));
#9403=DIRECTION('center_axis',(0.,-1.1019100660974E-16,1.));
#9404=DIRECTION('ref_axis',(0.,-1.,-1.1019100660974E-16));
#9405=DIRECTION('',(-1.,0.,0.));
#9406=DIRECTION('',(0.,1.,1.1019100660974E-16));
#9407=DIRECTION('center_axis',(0.,-1.,0.));
#9408=DIRECTION('ref_axis',(0.,0.,-1.));
#9409=DIRECTION('',(-1.,0.,0.));
#9410=DIRECTION('',(0.,0.,1.));
#9411=DIRECTION('center_axis',(0.,9.18258388414501E-17,-1.));
#9412=DIRECTION('ref_axis',(0.,1.,9.18258388414501E-17));
#9413=DIRECTION('',(0.,-1.,-9.18258388414501E-17));
#9414=DIRECTION('center_axis',(1.,0.,0.));
#9415=DIRECTION('ref_axis',(0.,0.,-1.));
#9416=DIRECTION('center_axis',(-1.,0.,0.));
#9417=DIRECTION('ref_axis',(0.,0.,1.));
#9418=DIRECTION('',(0.,-0.224951054343867,0.974370064785235));
#9419=DIRECTION('',(0.,0.974370064785235,0.224951054343868));
#9420=DIRECTION('',(0.,-0.974370064785235,-0.224951054343868));
#9421=DIRECTION('',(0.,-0.974370064785235,-0.224951054343868));
#9422=DIRECTION('',(0.,0.224951054343868,-0.974370064785235));
#9423=DIRECTION('',(0.,-0.974370064785235,-0.224951054343868));
#9424=DIRECTION('center_axis',(0.,-0.224951054343868,0.974370064785235));
#9425=DIRECTION('ref_axis',(0.,-0.974370064785235,-0.224951054343868));
#9426=DIRECTION('',(0.,-0.974370064785235,-0.224951054343868));
#9427=DIRECTION('',(-1.,0.,0.));
#9428=DIRECTION('center_axis',(1.,0.,0.));
#9429=DIRECTION('ref_axis',(0.,0.,-1.));
#9430=DIRECTION('',(0.,0.974370064785235,0.224951054343868));
#9431=DIRECTION('',(0.,-0.224951054343867,0.974370064785235));
#9432=DIRECTION('',(0.,-0.974370064785235,-0.224951054343868));
#9433=DIRECTION('',(0.,-0.224951054343868,0.974370064785235));
#9434=DIRECTION('',(0.,-0.974370064785235,-0.224951054343868));
#9435=DIRECTION('center_axis',(0.,0.224951054343868,-0.974370064785235));
#9436=DIRECTION('ref_axis',(0.,0.974370064785235,0.224951054343868));
#9437=DIRECTION('center_axis',(0.,0.974370064785235,0.224951054343868));
#9438=DIRECTION('ref_axis',(0.,-0.224951054343868,0.974370064785235));
#9439=DIRECTION('',(-1.,0.,0.));
#9440=DIRECTION('center_axis',(0.,-0.974370064785235,-0.224951054343867));
#9441=DIRECTION('ref_axis',(0.,0.224951054343867,-0.974370064785235));
#9442=DIRECTION('',(-1.,0.,0.));
#9443=DIRECTION('',(-1.,0.,0.));
#9444=DIRECTION('center_axis',(0.,-0.224951054343868,0.974370064785235));
#9445=DIRECTION('ref_axis',(0.,-0.974370064785235,-0.224951054343868));
#9446=DIRECTION('center_axis',(0.,0.224951054343868,-0.974370064785235));
#9447=DIRECTION('ref_axis',(0.,0.974370064785235,0.224951054343868));
#12176=CARTESIAN_POINT('',(0.,0.,0.));
#12177=CARTESIAN_POINT('Origin',(0.,40.8397926572471,-1.59119787916534));
#12178=CARTESIAN_POINT('',(-1.22464679914735E-16,39.3677205542196,9.23045840289062));
#12179=CARTESIAN_POINT('Origin',(0.,38.3933504894344,9.00550734854675));
#12180=CARTESIAN_POINT('',(-1.22464679914735E-16,41.1779050581859,1.3896878959578));
#12181=CARTESIAN_POINT('',(-1.22464679914735E-16,41.8141627220323,-1.36624682482147));
#12182=CARTESIAN_POINT('Origin',(0.,40.2035349934007,1.16473684161393));
#12183=CARTESIAN_POINT('Origin',(-20.6306248908449,20.2436822747633,-12.1953723836195));
#12184=CARTESIAN_POINT('',(-20.6306248908449,20.5804821002219,-6.98609547817754));
#12185=CARTESIAN_POINT('Origin',(-20.6306248908449,19.118927003044,-7.32352205969334));
#12186=CARTESIAN_POINT('',(-20.6306248908449,17.2062162850639,7.629455493601));
#12187=CARTESIAN_POINT('',(-20.6306248908449,21.7052373719412,-11.8579458021037));
#12188=CARTESIAN_POINT('Origin',(-20.6306248908449,15.744661187886,7.29202891208519));
#12189=CARTESIAN_POINT('Origin',(0.,17.5,19.325));
#12190=CARTESIAN_POINT('',(1.5,17.5,-3.675));
#12191=CARTESIAN_POINT('Origin',(0.,17.5,-3.675));
#12192=CARTESIAN_POINT('',(1.5,17.5,-17.4355957741627));
#12193=CARTESIAN_POINT('',(1.5,17.5,19.325));
#12194=CARTESIAN_POINT('Origin',(0.,17.5,-17.4355957741627));
#12195=CARTESIAN_POINT('Origin',(0.,17.5,19.325));
#12196=CARTESIAN_POINT('',(1.5,17.5,17.4355957741627));
#12197=CARTESIAN_POINT('Origin',(0.,17.5,17.4355957741627));
#12198=CARTESIAN_POINT('',(1.5,17.5,3.675));
#12199=CARTESIAN_POINT('',(1.5,17.5,19.325));
#12200=CARTESIAN_POINT('Origin',(0.,17.5,3.675));
#12201=CARTESIAN_POINT('Origin',(0.,17.5,0.));
#12202=CARTESIAN_POINT('',(17.1097742533325,17.5,-3.675));
#12203=CARTESIAN_POINT('Origin',(0.,17.5,0.));
#12204=CARTESIAN_POINT('',(-16.,11.4382861334438,-3.675));
#12205=CARTESIAN_POINT('Origin',(0.,17.5,-3.675));
#12206=CARTESIAN_POINT('',(-16.,11.4382861334438,3.675));
#12207=CARTESIAN_POINT('Origin',(-16.,17.5,0.));
#12208=CARTESIAN_POINT('',(17.1097742533325,17.5,3.675));
#12209=CARTESIAN_POINT('Origin',(0.,17.5,3.675));
#12210=CARTESIAN_POINT('Origin',(0.,17.5,0.));
#12211=CARTESIAN_POINT('',(16.5215428428775,21.9478081220939,3.675));
#12212=CARTESIAN_POINT('Origin',(0.,17.5,3.675));
#12213=CARTESIAN_POINT('',(16.5215428428775,21.9478081220939,-3.675));
#12214=CARTESIAN_POINT('Origin',(0.,21.9478081220939,0.));
#12215=CARTESIAN_POINT('Origin',(0.,17.5,-3.675));
#12216=CARTESIAN_POINT('',(-2.14861257031475,34.7331056821866,-2.15720480466577));
#12217=CARTESIAN_POINT('',(-2.14861257031475,32.0433564423134,9.49337913571913));
#12218=CARTESIAN_POINT('Origin',(-2.14861257031475,17.5,0.));
#12219=CARTESIAN_POINT('',(2.14861257031475,34.7331056821866,-2.15720480466577));
#12220=CARTESIAN_POINT('Origin',(0.,18.8448746199366,-5.82529197019245));
#12221=CARTESIAN_POINT('',(2.14861257031475,32.0433564423134,9.49337913571913));
#12222=CARTESIAN_POINT('Origin',(2.14861257031475,17.5,0.));
#12223=CARTESIAN_POINT('Origin',(0.,16.1551253800634,5.82529197019245));
#12224=CARTESIAN_POINT('',(-15.2970585407784,23.08461316672,-6.4079712685138));
#12225=CARTESIAN_POINT('',(-15.2970585407784,19.7103473515619,8.20757970326472));
#12226=CARTESIAN_POINT('Origin',(0.,21.3974802591409,0.899804217375471));
#12227=CARTESIAN_POINT('',(-15.2970585407784,11.9153868332801,6.4079712685138));
#12228=CARTESIAN_POINT('Origin',(0.,15.812867092421,7.30777548588927));
#12229=CARTESIAN_POINT('',(-15.2970585407784,15.2896526484381,-8.20757970326472));
#12230=CARTESIAN_POINT('Origin',(0.,13.6025197408591,-0.89980421737547));
#12231=CARTESIAN_POINT('Origin',(0.,19.187132907579,-7.30777548588926));
#12232=CARTESIAN_POINT('Origin',(0.,39.9993294599633,9.2345728386573));
#12233=CARTESIAN_POINT('',(-2.14861257031475,39.9682699940902,9.369106165755));
#12234=CARTESIAN_POINT('',(2.14861257031475,39.9682699940902,9.369106165755));
#12235=CARTESIAN_POINT('',(0.,39.9682699940902,9.369106165755));
#12236=CARTESIAN_POINT('',(-2.14861257031475,39.540006934909,11.2241172744453));
#12237=CARTESIAN_POINT('',(-2.14861257031475,42.2297561747823,-0.426466665939627));
#12238=CARTESIAN_POINT('',(2.14861257031475,39.540006934909,11.2241172744453));
#12239=CARTESIAN_POINT('',(-2.14861257031475,39.540006934909,11.2241172744453));
#12240=CARTESIAN_POINT('',(2.14861257031475,42.2297561747823,-0.426466665939627));
#12241=CARTESIAN_POINT('Origin',(-23.,20.5119281642586,4.73555175177994));
#12242=CARTESIAN_POINT('',(-23.,23.08461316672,-6.4079712685138));
#12243=CARTESIAN_POINT('',(-23.,23.08461316672,-6.4079712685138));
#12244=CARTESIAN_POINT('',(-23.,19.7103473515619,8.20757970326472));
#12245=CARTESIAN_POINT('',(-23.,20.5119281642586,4.73555175177994));
#12246=CARTESIAN_POINT('',(-23.,19.7103473515619,8.20757970326472));
#12247=CARTESIAN_POINT('Origin',(-23.,2.57268500246128,-11.1435230202937));
#12248=CARTESIAN_POINT('',(-23.,15.2896526484381,-8.20757970326472));
#12249=CARTESIAN_POINT('',(-23.,15.2896526484381,-8.20757970326472));
#12250=CARTESIAN_POINT('',(-23.,2.57268500246128,-11.1435230202937));
#12251=CARTESIAN_POINT('Origin',(-23.,12.7169676459768,2.935943317029));
#12252=CARTESIAN_POINT('',(-23.,11.9153868332801,6.4079712685138));
#12253=CARTESIAN_POINT('',(-23.,11.9153868332801,6.4079712685138));
#12254=CARTESIAN_POINT('',(-23.,12.7169676459768,2.935943317029));
#12255=CARTESIAN_POINT('Origin',(-23.,-0.801580812696699,3.47202795148484));
#12256=CARTESIAN_POINT('',(-23.,-0.801580812696699,3.47202795148484));
#12257=CARTESIAN_POINT('Origin',(-23.,0.,0.));
#12258=CARTESIAN_POINT('Origin',(25.,21.9478081220939,-3.675));
#12259=CARTESIAN_POINT('',(-16.,21.9478081220939,-3.675));
#12260=CARTESIAN_POINT('',(25.,21.9478081220939,-3.675));
#12261=CARTESIAN_POINT('',(-16.,21.9478081220939,-3.675));
#12262=CARTESIAN_POINT('Origin',(25.,21.9478081220939,3.675));
#12263=CARTESIAN_POINT('',(-16.,21.9478081220939,3.675));
#12264=CARTESIAN_POINT('',(25.,21.9478081220939,3.675));
#12265=CARTESIAN_POINT('',(-16.,21.9478081220939,3.675));
#12266=CARTESIAN_POINT('Origin',(25.,21.9478081220939,3.675));
#12267=CARTESIAN_POINT('',(-16.,21.9478081220939,3.675));
#12268=CARTESIAN_POINT('Origin',(-16.,0.,0.));
#12269=CARTESIAN_POINT('Origin',(2.14861257031475,42.2297561747823,-0.426466665939627));
#12270=CARTESIAN_POINT('',(2.14861257031475,37.1837280639145,0.467559478255006));
#12271=CARTESIAN_POINT('',(2.14861257031475,35.3735435599482,8.30832998518782));
#12272=CARTESIAN_POINT('',(2.14861257031475,37.6350297406403,-1.4872428465068));
#12273=CARTESIAN_POINT('',(2.14861257031475,39.9682699940902,9.369106165755));
#12274=CARTESIAN_POINT('',(2.14861257031475,39.540006934909,11.2241172744453));
#12275=CARTESIAN_POINT('',(2.14861257031475,42.2297561747823,-0.426466665939627));
#12276=CARTESIAN_POINT('',(2.14861257031475,42.2297561747823,-0.426466665939627));
#12277=CARTESIAN_POINT('',(2.14861257031475,41.7784544980564,1.52833565882218));
#12278=CARTESIAN_POINT('',(2.14861257031475,42.2297561747823,-0.426466665939627));
#12279=CARTESIAN_POINT('',(2.14861257031475,41.7784544980564,1.52833565882218));
#12280=CARTESIAN_POINT('Origin',(-2.14861257031475,42.2297561747823,-0.426466665939627));
#12281=CARTESIAN_POINT('',(-2.14861257031475,42.2297561747823,-0.426466665939627));
#12282=CARTESIAN_POINT('',(-2.14861257031475,42.2297561747823,-0.426466665939627));
#12283=CARTESIAN_POINT('',(-2.14861257031475,42.2297561747823,-0.426466665939627));
#12284=CARTESIAN_POINT('Origin',(-2.14861257031475,42.2297561747823,-0.426466665939627));
#12285=CARTESIAN_POINT('',(-2.14861257031475,35.3735435599482,8.30832998518782));
#12286=CARTESIAN_POINT('',(-2.14861257031475,35.3735435599482,8.30832998518782));
#12287=CARTESIAN_POINT('',(-2.14861257031475,37.1837280639145,0.467559478255006));
#12288=CARTESIAN_POINT('',(-2.14861257031475,37.1837280639145,0.467559478255006));
#12289=CARTESIAN_POINT('',(-2.14861257031475,41.7784544980564,1.52833565882219));
#12290=CARTESIAN_POINT('',(-2.14861257031475,41.7784544980564,1.52833565882219));
#12291=CARTESIAN_POINT('',(-2.14861257031475,42.2297561747823,-0.426466665939627));
#12292=CARTESIAN_POINT('',(-2.14861257031475,39.540006934909,11.2241172744453));
#12293=CARTESIAN_POINT('Origin',(-2.14861257031475,39.540006934909,11.2241172744453));
#12294=CARTESIAN_POINT('Origin',(0.,39.9993294599633,9.2345728386573));
#12295=CARTESIAN_POINT('',(0.,41.7784544980564,1.52833565882218));
#12296=CARTESIAN_POINT('Origin',(7.85138742968525,37.1837280639145,0.467559478255006));
#12297=CARTESIAN_POINT('',(7.85138742968525,37.1837280639145,0.467559478255006));
#12298=CARTESIAN_POINT('',(7.85138742968525,35.3735435599482,8.30832998518782));
#12299=CARTESIAN_POINT('Origin',(7.85138742968525,35.3735435599482,8.30832998518782));
#12300=CARTESIAN_POINT('Origin',(7.85138742968525,41.7784544980564,1.52833565882219));
#13166=UNCERTAINTY_MEASURE_WITH_UNIT(LENGTH_MEASURE(0.01),#13200,
'DISTANCE_ACCURACY_VALUE',
'Maximum model space distance between geometric entities at asserted c
onnectivities');
#13173=UNCERTAINTY_MEASURE_WITH_UNIT(LENGTH_MEASURE(0.01),#13200,
'DISTANCE_ACCURACY_VALUE',
'Maximum model space distance between geometric entities at asserted c
onnectivities');
#13192=(
GEOMETRIC_REPRESENTATION_CONTEXT(3)
GLOBAL_UNCERTAINTY_ASSIGNED_CONTEXT((#13166))
GLOBAL_UNIT_ASSIGNED_CONTEXT((#13200,#13202,#13203))
REPRESENTATION_CONTEXT('','3D')
);
#13199=(
GEOMETRIC_REPRESENTATION_CONTEXT(3)
GLOBAL_UNCERTAINTY_ASSIGNED_CONTEXT((#13173))
GLOBAL_UNIT_ASSIGNED_CONTEXT((#13200,#13202,#13203))
REPRESENTATION_CONTEXT('','3D')
);
#13200=(
LENGTH_UNIT()
NAMED_UNIT(*)
SI_UNIT(.MILLI.,.METRE.)
);
#13202=(
NAMED_UNIT(*)
PLANE_ANGLE_UNIT()
SI_UNIT($,.RADIAN.)
);
#13203=(
NAMED_UNIT(*)
SI_UNIT($,.STERADIAN.)
SOLID_ANGLE_UNIT()
);
#13222=SHAPE_DEFINITION_REPRESENTATION(#13261,#13296);
#13261=PRODUCT_DEFINITION_SHAPE('',$,#13322);
#13296=SHAPE_REPRESENTATION('',(#7618),#13192);
#13303=PRODUCT_DEFINITION_CONTEXT('part definition',#13380,'design');
#13322=PRODUCT_DEFINITION('Thumb Joint','Thumb Joint',#13347,#13303);
#13347=PRODUCT_DEFINITION_FORMATION('',$,#13400);
#13380=APPLICATION_CONTEXT(
'Core Data for Automotive Mechanical Design Process');
#13381=PRODUCT_CONTEXT('part definition',#13380,'mechanical');
#13400=PRODUCT('Thumb Joint','Thumb Joint',$,(#13381));
#13410=PRESENTATION_STYLE_ASSIGNMENT((#13415));
#13415=SURFACE_STYLE_USAGE(.BOTH.,#13420);
#13420=SURFACE_SIDE_STYLE('',(#13425));
#13425=SURFACE_STYLE_FILL_AREA(#13430);
#13430=FILL_AREA_STYLE('Opaque(227,224,212)',(#13435));
#13435=FILL_AREA_STYLE_COLOUR('Opaque(227,224,212)',#13440);
#13440=COLOUR_RGB('Opaque(227,224,212)',0.890196078431372,0.87843137254902,
0.831372549019608);
ENDSEC;
END-ISO-10303-21;
